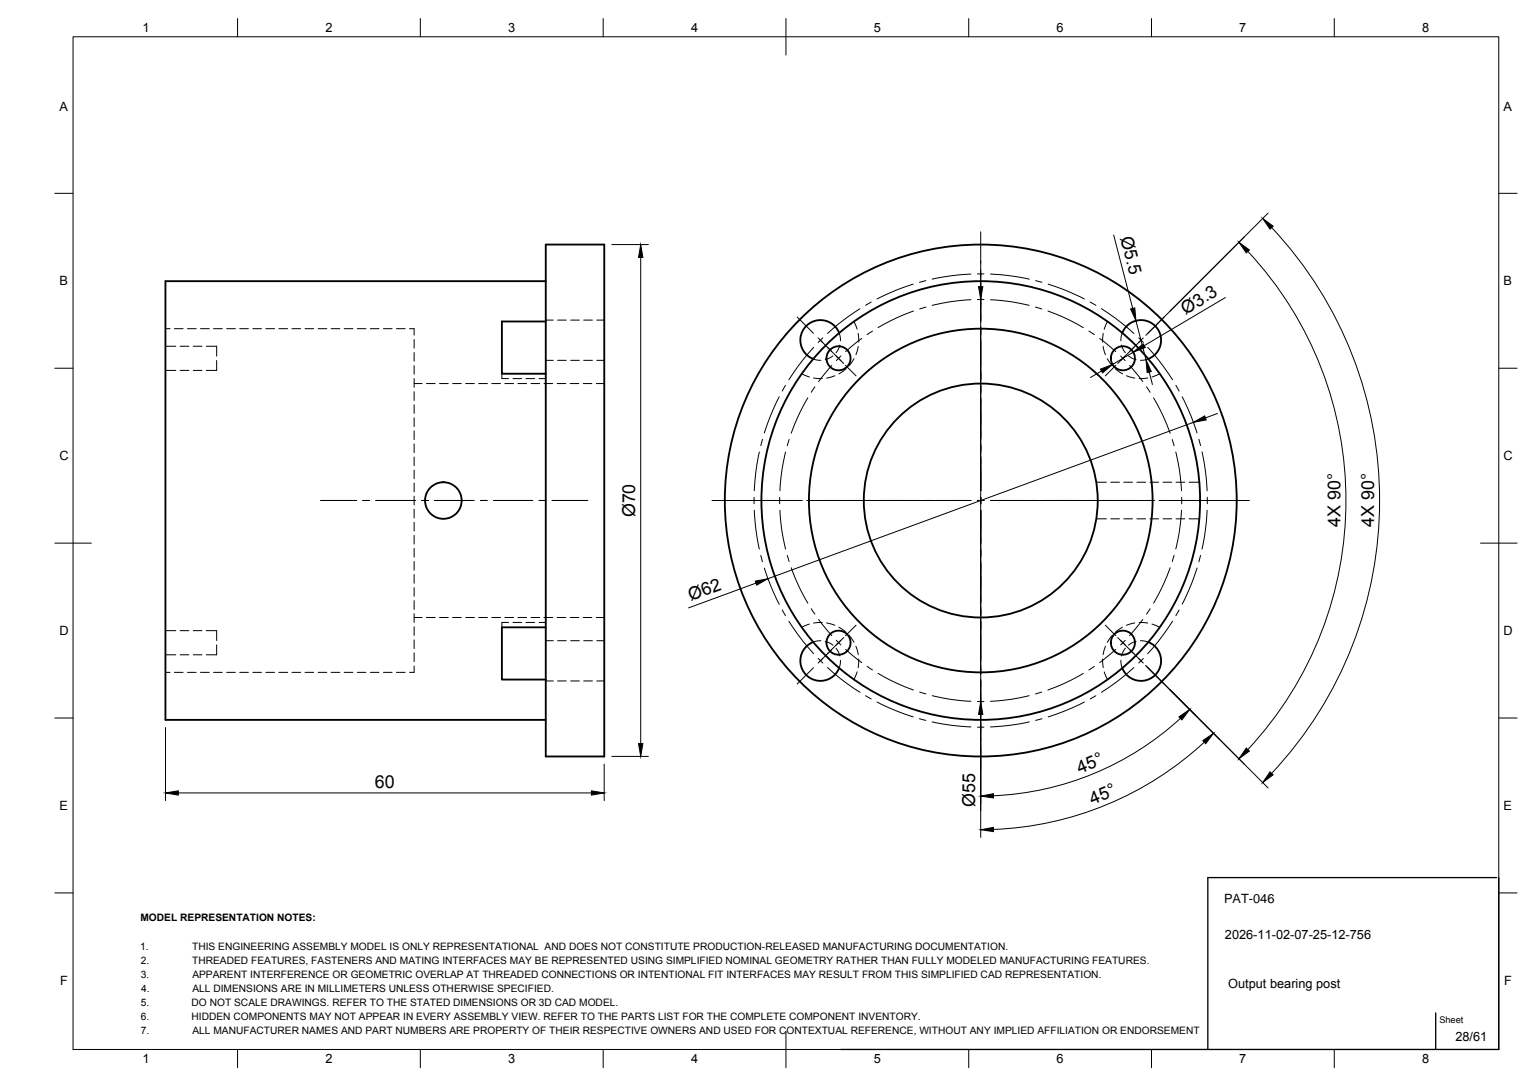
ISO-10303-21;
HEADER;
/* Generated by software containing ST-Developer
 * from STEP Tools, Inc. (www.steptools.com) 
 */

FILE_DESCRIPTION(
/* description */ ('Gear mesh backlash fixture'),
/* implementation_level */ '2;1');

FILE_NAME(
/* name */ 'Output bearing post.step',
/* time_stamp */ '2026-10-28T03:26:00-07:00',
/* author */ (''),
/* organization */ (''),
/* preprocessor_version */ 'ST-DEVELOPER v20.2',
/* originating_system */ 'Autodesk Translation Framework v15.17.0.0',
/* authorisation */ '');

FILE_SCHEMA (('AUTOMOTIVE_DESIGN { 1 0 10303 214 3 1 1 }'));
ENDSEC;

DATA;
#10=MECHANICAL_DESIGN_GEOMETRIC_PRESENTATION_REPRESENTATION('',(#1043),#57900);
#805=B_SPLINE_CURVE_WITH_KNOTS('',3,(#20786,#20787,#20788,#20789,#20790,
#20791,#20792,#20793,#20794,#20795),.UNSPECIFIED.,.F.,.F.,(4,2,2,2,4),(0.,
0.0943388977190341,0.188677795438068,0.283014752973434,0.377351710508801),
 .UNSPECIFIED.);
#806=B_SPLINE_CURVE_WITH_KNOTS('',3,(#20796,#20797,#20798,#20799,#20800,
#20801,#20802,#20803,#20804,#20805,#20806,#20807,#20808,#20809,#20810,#20811,
#20812,#20813,#20814,#20815,#20816,#20817,#20818,#20819,#20820,#20821),
 .UNSPECIFIED.,.F.,.F.,(4,2,2,2,2,2,2,2,2,2,2,2,4),(0.377351710508801,0.471688668044167,
0.566025625579534,0.660364523298568,0.754703421017602,0.849042318736636,
0.94338121645567,1.03771817399104,1.1320551315264,1.22639208906177,1.32072904659714,
1.41506794431617,1.5094068420352),.UNSPECIFIED.);
#807=B_SPLINE_CURVE_WITH_KNOTS('',3,(#20825,#20826,#20827,#20828,#20829,
#20830,#20831,#20832,#20833,#20834,#20835,#20836,#20837,#20838,#20839,#20840,
#20841,#20842,#20843,#20844,#20845,#20846,#20847,#20848,#20849,#20850),
 .UNSPECIFIED.,.F.,.F.,(4,2,2,2,2,2,2,2,2,2,2,2,4),(0.,0.0942186410044056,
0.188437282008811,0.282655768798836,0.376874255588861,0.471092742378886,
0.565311229168911,0.659529870173316,0.753748511177722,0.847967152182128,
0.942185793186533,1.03640427997656,1.13062276676658),.UNSPECIFIED.);
#808=B_SPLINE_CURVE_WITH_KNOTS('',3,(#20851,#20852,#20853,#20854,#20855,
#20856,#20857,#20858,#20859,#20860),.UNSPECIFIED.,.F.,.F.,(4,2,2,2,4),(1.13062276676658,
1.22484125355661,1.31905974034663,1.41327838135104,1.50749702235544),
 .UNSPECIFIED.);
#936=SHAPE_REPRESENTATION_RELATIONSHIP('SRR','None',#58133,#986);
#986=ADVANCED_BREP_SHAPE_REPRESENTATION('',(#1107),#57866);
#1043=STYLED_ITEM('',(#58465),#1107);
#1107=MANIFOLD_SOLID_BREP('Body1',#13604);
#1246=FACE_BOUND('',#2820,.T.);
#1247=FACE_BOUND('',#2821,.T.);
#1248=FACE_BOUND('',#2822,.T.);
#1249=FACE_BOUND('',#2823,.T.);
#1250=FACE_BOUND('',#2824,.T.);
#1251=FACE_BOUND('',#2829,.T.);
#1252=FACE_BOUND('',#2832,.T.);
#1253=FACE_BOUND('',#2835,.T.);
#1254=FACE_BOUND('',#2837,.T.);
#1255=FACE_BOUND('',#2838,.T.);
#1256=FACE_BOUND('',#2839,.T.);
#1257=FACE_BOUND('',#2840,.T.);
#1258=FACE_BOUND('',#2841,.T.);
#1259=FACE_BOUND('',#2843,.T.);
#1260=FACE_BOUND('',#2844,.T.);
#1261=FACE_BOUND('',#2845,.T.);
#1262=FACE_BOUND('',#2846,.T.);
#1263=FACE_BOUND('',#2847,.T.);
#1458=PLANE('',#14706);
#1459=PLANE('',#14710);
#1460=PLANE('',#14714);
#1461=PLANE('',#14718);
#1462=PLANE('',#14722);
#1463=PLANE('',#14727);
#1464=PLANE('',#14732);
#1465=PLANE('',#14737);
#1466=PLANE('',#14742);
#1467=PLANE('',#14763);
#1468=PLANE('',#14769);
#1469=PLANE('',#14770);
#1933=FACE_OUTER_BOUND('',#2801,.T.);
#1934=FACE_OUTER_BOUND('',#2802,.T.);
#1935=FACE_OUTER_BOUND('',#2803,.T.);
#1936=FACE_OUTER_BOUND('',#2804,.T.);
#1937=FACE_OUTER_BOUND('',#2805,.T.);
#1938=FACE_OUTER_BOUND('',#2806,.T.);
#1939=FACE_OUTER_BOUND('',#2807,.T.);
#1940=FACE_OUTER_BOUND('',#2808,.T.);
#1941=FACE_OUTER_BOUND('',#2809,.T.);
#1942=FACE_OUTER_BOUND('',#2810,.T.);
#1943=FACE_OUTER_BOUND('',#2811,.T.);
#1944=FACE_OUTER_BOUND('',#2812,.T.);
#1945=FACE_OUTER_BOUND('',#2813,.T.);
#1946=FACE_OUTER_BOUND('',#2814,.T.);
#1947=FACE_OUTER_BOUND('',#2815,.T.);
#1948=FACE_OUTER_BOUND('',#2816,.T.);
#1949=FACE_OUTER_BOUND('',#2817,.T.);
#1950=FACE_OUTER_BOUND('',#2818,.T.);
#1951=FACE_OUTER_BOUND('',#2819,.T.);
#1952=FACE_OUTER_BOUND('',#2825,.T.);
#1953=FACE_OUTER_BOUND('',#2826,.T.);
#1954=FACE_OUTER_BOUND('',#2827,.T.);
#1955=FACE_OUTER_BOUND('',#2828,.T.);
#1956=FACE_OUTER_BOUND('',#2830,.T.);
#1957=FACE_OUTER_BOUND('',#2831,.T.);
#1958=FACE_OUTER_BOUND('',#2833,.T.);
#1959=FACE_OUTER_BOUND('',#2834,.T.);
#1960=FACE_OUTER_BOUND('',#2836,.T.);
#1961=FACE_OUTER_BOUND('',#2842,.T.);
#2801=EDGE_LOOP('',(#9947,#9948,#9949,#9950,#9951,#9952));
#2802=EDGE_LOOP('',(#9953,#9954,#9955,#9956));
#2803=EDGE_LOOP('',(#9957));
#2804=EDGE_LOOP('',(#9958,#9959,#9960,#9961));
#2805=EDGE_LOOP('',(#9962));
#2806=EDGE_LOOP('',(#9963,#9964,#9965,#9966));
#2807=EDGE_LOOP('',(#9967));
#2808=EDGE_LOOP('',(#9968,#9969,#9970,#9971));
#2809=EDGE_LOOP('',(#9972));
#2810=EDGE_LOOP('',(#9973,#9974,#9975,#9976));
#2811=EDGE_LOOP('',(#9977,#9978));
#2812=EDGE_LOOP('',(#9979,#9980,#9981,#9982));
#2813=EDGE_LOOP('',(#9983,#9984));
#2814=EDGE_LOOP('',(#9985,#9986,#9987,#9988));
#2815=EDGE_LOOP('',(#9989,#9990));
#2816=EDGE_LOOP('',(#9991,#9992,#9993,#9994));
#2817=EDGE_LOOP('',(#9995,#9996));
#2818=EDGE_LOOP('',(#9997,#9998,#9999,#10000));
#2819=EDGE_LOOP('',(#10001));
#2820=EDGE_LOOP('',(#10002,#10003,#10004,#10005,#10006,#10007,#10008,#10009,
#10010));
#2821=EDGE_LOOP('',(#10011));
#2822=EDGE_LOOP('',(#10012));
#2823=EDGE_LOOP('',(#10013));
#2824=EDGE_LOOP('',(#10014));
#2825=EDGE_LOOP('',(#10015,#10016,#10017,#10018));
#2826=EDGE_LOOP('',(#10019,#10020,#10021,#10022));
#2827=EDGE_LOOP('',(#10023,#10024,#10025,#10026));
#2828=EDGE_LOOP('',(#10027,#10028,#10029,#10030,#10031,#10032,#10033,#10034,
#10035,#10036,#10037,#10038,#10039,#10040,#10041,#10042,#10043,#10044,#10045,
#10046));
#2829=EDGE_LOOP('',(#10047,#10048));
#2830=EDGE_LOOP('',(#10049,#10050,#10051,#10052));
#2831=EDGE_LOOP('',(#10053));
#2832=EDGE_LOOP('',(#10054));
#2833=EDGE_LOOP('',(#10055,#10056,#10057,#10058));
#2834=EDGE_LOOP('',(#10059,#10060,#10061,#10062));
#2835=EDGE_LOOP('',(#10063,#10064));
#2836=EDGE_LOOP('',(#10065));
#2837=EDGE_LOOP('',(#10066));
#2838=EDGE_LOOP('',(#10067));
#2839=EDGE_LOOP('',(#10068));
#2840=EDGE_LOOP('',(#10069));
#2841=EDGE_LOOP('',(#10070));
#2842=EDGE_LOOP('',(#10071));
#2843=EDGE_LOOP('',(#10072));
#2844=EDGE_LOOP('',(#10073));
#2845=EDGE_LOOP('',(#10074));
#2846=EDGE_LOOP('',(#10075));
#2847=EDGE_LOOP('',(#10076));
#3686=LINE('',#20823,#4575);
#3687=LINE('',#20865,#4576);
#3688=LINE('',#20872,#4577);
#3689=LINE('',#20879,#4578);
#3690=LINE('',#20886,#4579);
#3691=LINE('',#20892,#4580);
#3692=LINE('',#20896,#4581);
#3693=LINE('',#20903,#4582);
#3694=LINE('',#20907,#4583);
#3695=LINE('',#20914,#4584);
#3696=LINE('',#20918,#4585);
#3697=LINE('',#20925,#4586);
#3698=LINE('',#20929,#4587);
#3699=LINE('',#20937,#4588);
#3700=LINE('',#20957,#4589);
#3701=LINE('',#20961,#4590);
#3702=LINE('',#20965,#4591);
#3703=LINE('',#20969,#4592);
#3704=LINE('',#20974,#4593);
#3705=LINE('',#20981,#4594);
#3706=LINE('',#20985,#4595);
#4575=VECTOR('',#16869,0.25);
#4576=VECTOR('',#16874,0.165);
#4577=VECTOR('',#16883,0.165);
#4578=VECTOR('',#16892,0.164999999999999);
#4579=VECTOR('',#16901,0.165);
#4580=VECTOR('',#16908,1.);
#4581=VECTOR('',#16911,1.);
#4582=VECTOR('',#16920,1.);
#4583=VECTOR('',#16923,1.);
#4584=VECTOR('',#16932,1.);
#4585=VECTOR('',#16935,1.);
#4586=VECTOR('',#16944,1.);
#4587=VECTOR('',#16947,1.);
#4588=VECTOR('',#16958,0.275);
#4589=VECTOR('',#16985,0.275);
#4590=VECTOR('',#16990,0.275);
#4591=VECTOR('',#16995,0.275);
#4592=VECTOR('',#17000,3.);
#4593=VECTOR('',#17005,2.35);
#4594=VECTOR('',#17014,3.5);
#4595=VECTOR('',#17019,1.6);
#5427=CIRCLE('',#14704,0.165);
#5428=CIRCLE('',#14705,0.165);
#5429=CIRCLE('',#14708,0.165);
#5430=CIRCLE('',#14709,0.165);
#5431=CIRCLE('',#14712,0.164999999999999);
#5432=CIRCLE('',#14713,0.164999999999999);
#5433=CIRCLE('',#14716,0.165);
#5434=CIRCLE('',#14717,0.165);
#5435=CIRCLE('',#14720,0.525);
#5436=CIRCLE('',#14721,0.525);
#5437=CIRCLE('',#14723,3.);
#5438=CIRCLE('',#14725,0.525);
#5439=CIRCLE('',#14726,0.525);
#5440=CIRCLE('',#14728,3.);
#5441=CIRCLE('',#14730,0.525);
#5442=CIRCLE('',#14731,0.525);
#5443=CIRCLE('',#14733,3.);
#5444=CIRCLE('',#14735,0.525);
#5445=CIRCLE('',#14736,0.525);
#5446=CIRCLE('',#14738,3.);
#5447=CIRCLE('',#14740,0.275);
#5448=CIRCLE('',#14741,0.275);
#5449=CIRCLE('',#14743,3.5);
#5450=CIRCLE('',#14744,3.);
#5451=CIRCLE('',#14745,3.);
#5452=CIRCLE('',#14746,3.);
#5453=CIRCLE('',#14747,3.);
#5454=CIRCLE('',#14748,3.);
#5455=CIRCLE('',#14749,0.275);
#5456=CIRCLE('',#14750,0.275);
#5457=CIRCLE('',#14751,0.275);
#5458=CIRCLE('',#14753,0.275);
#5459=CIRCLE('',#14755,0.275);
#5460=CIRCLE('',#14757,0.275);
#5461=CIRCLE('',#14759,3.);
#5462=CIRCLE('',#14761,2.35);
#5463=CIRCLE('',#14762,2.35);
#5464=CIRCLE('',#14764,1.6);
#5465=CIRCLE('',#14766,3.5);
#5466=CIRCLE('',#14768,1.6);
#6139=VERTEX_POINT('',#20784);
#6140=VERTEX_POINT('',#20785);
#6141=VERTEX_POINT('',#20822);
#6142=VERTEX_POINT('',#20824);
#6143=VERTEX_POINT('',#20862);
#6144=VERTEX_POINT('',#20864);
#6145=VERTEX_POINT('',#20869);
#6146=VERTEX_POINT('',#20871);
#6147=VERTEX_POINT('',#20876);
#6148=VERTEX_POINT('',#20878);
#6149=VERTEX_POINT('',#20883);
#6150=VERTEX_POINT('',#20885);
#6151=VERTEX_POINT('',#20890);
#6152=VERTEX_POINT('',#20891);
#6153=VERTEX_POINT('',#20893);
#6154=VERTEX_POINT('',#20895);
#6155=VERTEX_POINT('',#20901);
#6156=VERTEX_POINT('',#20902);
#6157=VERTEX_POINT('',#20904);
#6158=VERTEX_POINT('',#20906);
#6159=VERTEX_POINT('',#20912);
#6160=VERTEX_POINT('',#20913);
#6161=VERTEX_POINT('',#20915);
#6162=VERTEX_POINT('',#20917);
#6163=VERTEX_POINT('',#20923);
#6164=VERTEX_POINT('',#20924);
#6165=VERTEX_POINT('',#20926);
#6166=VERTEX_POINT('',#20928);
#6167=VERTEX_POINT('',#20934);
#6168=VERTEX_POINT('',#20936);
#6169=VERTEX_POINT('',#20940);
#6170=VERTEX_POINT('',#20942);
#6171=VERTEX_POINT('',#20948);
#6172=VERTEX_POINT('',#20950);
#6173=VERTEX_POINT('',#20952);
#6174=VERTEX_POINT('',#20955);
#6175=VERTEX_POINT('',#20959);
#6176=VERTEX_POINT('',#20963);
#6177=VERTEX_POINT('',#20967);
#6178=VERTEX_POINT('',#20971);
#6179=VERTEX_POINT('',#20973);
#6180=VERTEX_POINT('',#20977);
#6181=VERTEX_POINT('',#20980);
#6182=VERTEX_POINT('',#20984);
#7560=EDGE_CURVE('',#6139,#6140,#805,.T.);
#7561=EDGE_CURVE('',#6140,#6139,#806,.T.);
#7562=EDGE_CURVE('',#6140,#6141,#3686,.T.);
#7563=EDGE_CURVE('',#6142,#6141,#807,.T.);
#7564=EDGE_CURVE('',#6141,#6142,#808,.T.);
#7565=EDGE_CURVE('',#6143,#6143,#5427,.T.);
#7566=EDGE_CURVE('',#6143,#6144,#3687,.T.);
#7567=EDGE_CURVE('',#6144,#6144,#5428,.T.);
#7568=EDGE_CURVE('',#6145,#6145,#5429,.T.);
#7569=EDGE_CURVE('',#6145,#6146,#3688,.T.);
#7570=EDGE_CURVE('',#6146,#6146,#5430,.T.);
#7571=EDGE_CURVE('',#6147,#6147,#5431,.T.);
#7572=EDGE_CURVE('',#6147,#6148,#3689,.T.);
#7573=EDGE_CURVE('',#6148,#6148,#5432,.T.);
#7574=EDGE_CURVE('',#6149,#6149,#5433,.T.);
#7575=EDGE_CURVE('',#6149,#6150,#3690,.T.);
#7576=EDGE_CURVE('',#6150,#6150,#5434,.T.);
#7577=EDGE_CURVE('',#6151,#6152,#3691,.T.);
#7578=EDGE_CURVE('',#6151,#6153,#5435,.T.);
#7579=EDGE_CURVE('',#6154,#6153,#3692,.T.);
#7580=EDGE_CURVE('',#6152,#6154,#5436,.T.);
#7581=EDGE_CURVE('',#6153,#6151,#5437,.T.);
#7582=EDGE_CURVE('',#6155,#6156,#3693,.T.);
#7583=EDGE_CURVE('',#6155,#6157,#5438,.T.);
#7584=EDGE_CURVE('',#6158,#6157,#3694,.T.);
#7585=EDGE_CURVE('',#6156,#6158,#5439,.T.);
#7586=EDGE_CURVE('',#6157,#6155,#5440,.T.);
#7587=EDGE_CURVE('',#6159,#6160,#3695,.T.);
#7588=EDGE_CURVE('',#6159,#6161,#5441,.T.);
#7589=EDGE_CURVE('',#6162,#6161,#3696,.T.);
#7590=EDGE_CURVE('',#6160,#6162,#5442,.T.);
#7591=EDGE_CURVE('',#6161,#6159,#5443,.T.);
#7592=EDGE_CURVE('',#6163,#6164,#3697,.T.);
#7593=EDGE_CURVE('',#6163,#6165,#5444,.T.);
#7594=EDGE_CURVE('',#6166,#6165,#3698,.T.);
#7595=EDGE_CURVE('',#6164,#6166,#5445,.T.);
#7596=EDGE_CURVE('',#6165,#6163,#5446,.T.);
#7597=EDGE_CURVE('',#6167,#6167,#5447,.T.);
#7598=EDGE_CURVE('',#6167,#6168,#3699,.T.);
#7599=EDGE_CURVE('',#6168,#6168,#5448,.T.);
#7600=EDGE_CURVE('',#6169,#6169,#5449,.T.);
#7601=EDGE_CURVE('',#6156,#6170,#5450,.T.);
#7602=EDGE_CURVE('',#6160,#6158,#5451,.T.);
#7603=EDGE_CURVE('',#6164,#6162,#5452,.T.);
#7604=EDGE_CURVE('',#6152,#6166,#5453,.T.);
#7605=EDGE_CURVE('',#6170,#6154,#5454,.T.);
#7606=EDGE_CURVE('',#6171,#6171,#5455,.T.);
#7607=EDGE_CURVE('',#6172,#6172,#5456,.T.);
#7608=EDGE_CURVE('',#6173,#6173,#5457,.T.);
#7609=EDGE_CURVE('',#6174,#6174,#5458,.T.);
#7610=EDGE_CURVE('',#6174,#6172,#3700,.T.);
#7611=EDGE_CURVE('',#6175,#6175,#5459,.T.);
#7612=EDGE_CURVE('',#6175,#6171,#3701,.T.);
#7613=EDGE_CURVE('',#6176,#6176,#5460,.T.);
#7614=EDGE_CURVE('',#6176,#6173,#3702,.T.);
#7615=EDGE_CURVE('',#6177,#6177,#5461,.T.);
#7616=EDGE_CURVE('',#6177,#6170,#3703,.T.);
#7617=EDGE_CURVE('',#6178,#6178,#5462,.T.);
#7618=EDGE_CURVE('',#6178,#6179,#3704,.T.);
#7619=EDGE_CURVE('',#6179,#6179,#5463,.T.);
#7620=EDGE_CURVE('',#6180,#6180,#5464,.T.);
#7621=EDGE_CURVE('',#6169,#6181,#3705,.T.);
#7622=EDGE_CURVE('',#6181,#6181,#5465,.T.);
#7623=EDGE_CURVE('',#6180,#6182,#3706,.T.);
#7624=EDGE_CURVE('',#6182,#6182,#5466,.T.);
#9947=ORIENTED_EDGE('',*,*,#7560,.F.);
#9948=ORIENTED_EDGE('',*,*,#7561,.F.);
#9949=ORIENTED_EDGE('',*,*,#7562,.T.);
#9950=ORIENTED_EDGE('',*,*,#7563,.F.);
#9951=ORIENTED_EDGE('',*,*,#7564,.F.);
#9952=ORIENTED_EDGE('',*,*,#7562,.F.);
#9953=ORIENTED_EDGE('',*,*,#7565,.F.);
#9954=ORIENTED_EDGE('',*,*,#7566,.T.);
#9955=ORIENTED_EDGE('',*,*,#7567,.F.);
#9956=ORIENTED_EDGE('',*,*,#7566,.F.);
#9957=ORIENTED_EDGE('',*,*,#7565,.T.);
#9958=ORIENTED_EDGE('',*,*,#7568,.F.);
#9959=ORIENTED_EDGE('',*,*,#7569,.T.);
#9960=ORIENTED_EDGE('',*,*,#7570,.F.);
#9961=ORIENTED_EDGE('',*,*,#7569,.F.);
#9962=ORIENTED_EDGE('',*,*,#7568,.T.);
#9963=ORIENTED_EDGE('',*,*,#7571,.F.);
#9964=ORIENTED_EDGE('',*,*,#7572,.T.);
#9965=ORIENTED_EDGE('',*,*,#7573,.F.);
#9966=ORIENTED_EDGE('',*,*,#7572,.F.);
#9967=ORIENTED_EDGE('',*,*,#7571,.T.);
#9968=ORIENTED_EDGE('',*,*,#7574,.F.);
#9969=ORIENTED_EDGE('',*,*,#7575,.T.);
#9970=ORIENTED_EDGE('',*,*,#7576,.F.);
#9971=ORIENTED_EDGE('',*,*,#7575,.F.);
#9972=ORIENTED_EDGE('',*,*,#7574,.T.);
#9973=ORIENTED_EDGE('',*,*,#7577,.F.);
#9974=ORIENTED_EDGE('',*,*,#7578,.T.);
#9975=ORIENTED_EDGE('',*,*,#7579,.F.);
#9976=ORIENTED_EDGE('',*,*,#7580,.F.);
#9977=ORIENTED_EDGE('',*,*,#7581,.F.);
#9978=ORIENTED_EDGE('',*,*,#7578,.F.);
#9979=ORIENTED_EDGE('',*,*,#7582,.F.);
#9980=ORIENTED_EDGE('',*,*,#7583,.T.);
#9981=ORIENTED_EDGE('',*,*,#7584,.F.);
#9982=ORIENTED_EDGE('',*,*,#7585,.F.);
#9983=ORIENTED_EDGE('',*,*,#7586,.F.);
#9984=ORIENTED_EDGE('',*,*,#7583,.F.);
#9985=ORIENTED_EDGE('',*,*,#7587,.F.);
#9986=ORIENTED_EDGE('',*,*,#7588,.T.);
#9987=ORIENTED_EDGE('',*,*,#7589,.F.);
#9988=ORIENTED_EDGE('',*,*,#7590,.F.);
#9989=ORIENTED_EDGE('',*,*,#7591,.F.);
#9990=ORIENTED_EDGE('',*,*,#7588,.F.);
#9991=ORIENTED_EDGE('',*,*,#7592,.F.);
#9992=ORIENTED_EDGE('',*,*,#7593,.T.);
#9993=ORIENTED_EDGE('',*,*,#7594,.F.);
#9994=ORIENTED_EDGE('',*,*,#7595,.F.);
#9995=ORIENTED_EDGE('',*,*,#7596,.F.);
#9996=ORIENTED_EDGE('',*,*,#7593,.F.);
#9997=ORIENTED_EDGE('',*,*,#7597,.F.);
#9998=ORIENTED_EDGE('',*,*,#7598,.T.);
#9999=ORIENTED_EDGE('',*,*,#7599,.F.);
#10000=ORIENTED_EDGE('',*,*,#7598,.F.);
#10001=ORIENTED_EDGE('',*,*,#7600,.T.);
#10002=ORIENTED_EDGE('',*,*,#7601,.F.);
#10003=ORIENTED_EDGE('',*,*,#7585,.T.);
#10004=ORIENTED_EDGE('',*,*,#7602,.F.);
#10005=ORIENTED_EDGE('',*,*,#7590,.T.);
#10006=ORIENTED_EDGE('',*,*,#7603,.F.);
#10007=ORIENTED_EDGE('',*,*,#7595,.T.);
#10008=ORIENTED_EDGE('',*,*,#7604,.F.);
#10009=ORIENTED_EDGE('',*,*,#7580,.T.);
#10010=ORIENTED_EDGE('',*,*,#7605,.F.);
#10011=ORIENTED_EDGE('',*,*,#7606,.T.);
#10012=ORIENTED_EDGE('',*,*,#7599,.T.);
#10013=ORIENTED_EDGE('',*,*,#7607,.T.);
#10014=ORIENTED_EDGE('',*,*,#7608,.T.);
#10015=ORIENTED_EDGE('',*,*,#7609,.F.);
#10016=ORIENTED_EDGE('',*,*,#7610,.T.);
#10017=ORIENTED_EDGE('',*,*,#7607,.F.);
#10018=ORIENTED_EDGE('',*,*,#7610,.F.);
#10019=ORIENTED_EDGE('',*,*,#7611,.F.);
#10020=ORIENTED_EDGE('',*,*,#7612,.T.);
#10021=ORIENTED_EDGE('',*,*,#7606,.F.);
#10022=ORIENTED_EDGE('',*,*,#7612,.F.);
#10023=ORIENTED_EDGE('',*,*,#7613,.F.);
#10024=ORIENTED_EDGE('',*,*,#7614,.T.);
#10025=ORIENTED_EDGE('',*,*,#7608,.F.);
#10026=ORIENTED_EDGE('',*,*,#7614,.F.);
#10027=ORIENTED_EDGE('',*,*,#7615,.F.);
#10028=ORIENTED_EDGE('',*,*,#7616,.T.);
#10029=ORIENTED_EDGE('',*,*,#7605,.T.);
#10030=ORIENTED_EDGE('',*,*,#7579,.T.);
#10031=ORIENTED_EDGE('',*,*,#7581,.T.);
#10032=ORIENTED_EDGE('',*,*,#7577,.T.);
#10033=ORIENTED_EDGE('',*,*,#7604,.T.);
#10034=ORIENTED_EDGE('',*,*,#7594,.T.);
#10035=ORIENTED_EDGE('',*,*,#7596,.T.);
#10036=ORIENTED_EDGE('',*,*,#7592,.T.);
#10037=ORIENTED_EDGE('',*,*,#7603,.T.);
#10038=ORIENTED_EDGE('',*,*,#7589,.T.);
#10039=ORIENTED_EDGE('',*,*,#7591,.T.);
#10040=ORIENTED_EDGE('',*,*,#7587,.T.);
#10041=ORIENTED_EDGE('',*,*,#7602,.T.);
#10042=ORIENTED_EDGE('',*,*,#7584,.T.);
#10043=ORIENTED_EDGE('',*,*,#7586,.T.);
#10044=ORIENTED_EDGE('',*,*,#7582,.T.);
#10045=ORIENTED_EDGE('',*,*,#7601,.T.);
#10046=ORIENTED_EDGE('',*,*,#7616,.F.);
#10047=ORIENTED_EDGE('',*,*,#7563,.T.);
#10048=ORIENTED_EDGE('',*,*,#7564,.T.);
#10049=ORIENTED_EDGE('',*,*,#7617,.F.);
#10050=ORIENTED_EDGE('',*,*,#7618,.T.);
#10051=ORIENTED_EDGE('',*,*,#7619,.F.);
#10052=ORIENTED_EDGE('',*,*,#7618,.F.);
#10053=ORIENTED_EDGE('',*,*,#7617,.T.);
#10054=ORIENTED_EDGE('',*,*,#7620,.F.);
#10055=ORIENTED_EDGE('',*,*,#7600,.F.);
#10056=ORIENTED_EDGE('',*,*,#7621,.T.);
#10057=ORIENTED_EDGE('',*,*,#7622,.T.);
#10058=ORIENTED_EDGE('',*,*,#7621,.F.);
#10059=ORIENTED_EDGE('',*,*,#7620,.T.);
#10060=ORIENTED_EDGE('',*,*,#7623,.T.);
#10061=ORIENTED_EDGE('',*,*,#7624,.T.);
#10062=ORIENTED_EDGE('',*,*,#7623,.F.);
#10063=ORIENTED_EDGE('',*,*,#7560,.T.);
#10064=ORIENTED_EDGE('',*,*,#7561,.T.);
#10065=ORIENTED_EDGE('',*,*,#7615,.T.);
#10066=ORIENTED_EDGE('',*,*,#7619,.T.);
#10067=ORIENTED_EDGE('',*,*,#7576,.T.);
#10068=ORIENTED_EDGE('',*,*,#7573,.T.);
#10069=ORIENTED_EDGE('',*,*,#7570,.T.);
#10070=ORIENTED_EDGE('',*,*,#7567,.T.);
#10071=ORIENTED_EDGE('',*,*,#7622,.F.);
#10072=ORIENTED_EDGE('',*,*,#7624,.F.);
#10073=ORIENTED_EDGE('',*,*,#7609,.T.);
#10074=ORIENTED_EDGE('',*,*,#7597,.T.);
#10075=ORIENTED_EDGE('',*,*,#7613,.T.);
#10076=ORIENTED_EDGE('',*,*,#7611,.T.);
#12672=CYLINDRICAL_SURFACE('',#14702,0.25);
#12673=CYLINDRICAL_SURFACE('',#14703,0.165);
#12674=CYLINDRICAL_SURFACE('',#14707,0.165);
#12675=CYLINDRICAL_SURFACE('',#14711,0.164999999999999);
#12676=CYLINDRICAL_SURFACE('',#14715,0.165);
#12677=CYLINDRICAL_SURFACE('',#14719,0.525);
#12678=CYLINDRICAL_SURFACE('',#14724,0.525);
#12679=CYLINDRICAL_SURFACE('',#14729,0.525);
#12680=CYLINDRICAL_SURFACE('',#14734,0.525);
#12681=CYLINDRICAL_SURFACE('',#14739,0.275);
#12682=CYLINDRICAL_SURFACE('',#14752,0.275);
#12683=CYLINDRICAL_SURFACE('',#14754,0.275);
#12684=CYLINDRICAL_SURFACE('',#14756,0.275);
#12685=CYLINDRICAL_SURFACE('',#14758,3.);
#12686=CYLINDRICAL_SURFACE('',#14760,2.35);
#12687=CYLINDRICAL_SURFACE('',#14765,3.5);
#12688=CYLINDRICAL_SURFACE('',#14767,1.6);
#13050=ADVANCED_FACE('',(#1933),#12672,.F.);
#13051=ADVANCED_FACE('',(#1934),#12673,.F.);
#13052=ADVANCED_FACE('',(#1935),#1458,.T.);
#13053=ADVANCED_FACE('',(#1936),#12674,.F.);
#13054=ADVANCED_FACE('',(#1937),#1459,.T.);
#13055=ADVANCED_FACE('',(#1938),#12675,.F.);
#13056=ADVANCED_FACE('',(#1939),#1460,.T.);
#13057=ADVANCED_FACE('',(#1940),#12676,.F.);
#13058=ADVANCED_FACE('',(#1941),#1461,.T.);
#13059=ADVANCED_FACE('',(#1942),#12677,.F.);
#13060=ADVANCED_FACE('',(#1943),#1462,.F.);
#13061=ADVANCED_FACE('',(#1944),#12678,.F.);
#13062=ADVANCED_FACE('',(#1945),#1463,.F.);
#13063=ADVANCED_FACE('',(#1946),#12679,.F.);
#13064=ADVANCED_FACE('',(#1947),#1464,.F.);
#13065=ADVANCED_FACE('',(#1948),#12680,.F.);
#13066=ADVANCED_FACE('',(#1949),#1465,.F.);
#13067=ADVANCED_FACE('',(#1950),#12681,.F.);
#13068=ADVANCED_FACE('',(#1951,#1246,#1247,#1248,#1249,#1250),#1466,.T.);
#13069=ADVANCED_FACE('',(#1952),#12682,.F.);
#13070=ADVANCED_FACE('',(#1953),#12683,.F.);
#13071=ADVANCED_FACE('',(#1954),#12684,.F.);
#13072=ADVANCED_FACE('',(#1955,#1251),#12685,.T.);
#13073=ADVANCED_FACE('',(#1956),#12686,.F.);
#13074=ADVANCED_FACE('',(#1957,#1252),#1467,.T.);
#13075=ADVANCED_FACE('',(#1958),#12687,.T.);
#13076=ADVANCED_FACE('',(#1959,#1253),#12688,.F.);
#13077=ADVANCED_FACE('',(#1960,#1254,#1255,#1256,#1257,#1258),#1468,.T.);
#13078=ADVANCED_FACE('',(#1961,#1259,#1260,#1261,#1262,#1263),#1469,.F.);
#13604=CLOSED_SHELL('',(#13050,#13051,#13052,#13053,#13054,#13055,#13056,
#13057,#13058,#13059,#13060,#13061,#13062,#13063,#13064,#13065,#13066,#13067,
#13068,#13069,#13070,#13071,#13072,#13073,#13074,#13075,#13076,#13077,#13078));
#14701=AXIS2_PLACEMENT_3D('',#20782,#16865,#16866);
#14702=AXIS2_PLACEMENT_3D('',#20783,#16867,#16868);
#14703=AXIS2_PLACEMENT_3D('',#20861,#16870,#16871);
#14704=AXIS2_PLACEMENT_3D('',#20863,#16872,#16873);
#14705=AXIS2_PLACEMENT_3D('',#20866,#16875,#16876);
#14706=AXIS2_PLACEMENT_3D('',#20867,#16877,#16878);
#14707=AXIS2_PLACEMENT_3D('',#20868,#16879,#16880);
#14708=AXIS2_PLACEMENT_3D('',#20870,#16881,#16882);
#14709=AXIS2_PLACEMENT_3D('',#20873,#16884,#16885);
#14710=AXIS2_PLACEMENT_3D('',#20874,#16886,#16887);
#14711=AXIS2_PLACEMENT_3D('',#20875,#16888,#16889);
#14712=AXIS2_PLACEMENT_3D('',#20877,#16890,#16891);
#14713=AXIS2_PLACEMENT_3D('',#20880,#16893,#16894);
#14714=AXIS2_PLACEMENT_3D('',#20881,#16895,#16896);
#14715=AXIS2_PLACEMENT_3D('',#20882,#16897,#16898);
#14716=AXIS2_PLACEMENT_3D('',#20884,#16899,#16900);
#14717=AXIS2_PLACEMENT_3D('',#20887,#16902,#16903);
#14718=AXIS2_PLACEMENT_3D('',#20888,#16904,#16905);
#14719=AXIS2_PLACEMENT_3D('',#20889,#16906,#16907);
#14720=AXIS2_PLACEMENT_3D('',#20894,#16909,#16910);
#14721=AXIS2_PLACEMENT_3D('',#20897,#16912,#16913);
#14722=AXIS2_PLACEMENT_3D('',#20898,#16914,#16915);
#14723=AXIS2_PLACEMENT_3D('',#20899,#16916,#16917);
#14724=AXIS2_PLACEMENT_3D('',#20900,#16918,#16919);
#14725=AXIS2_PLACEMENT_3D('',#20905,#16921,#16922);
#14726=AXIS2_PLACEMENT_3D('',#20908,#16924,#16925);
#14727=AXIS2_PLACEMENT_3D('',#20909,#16926,#16927);
#14728=AXIS2_PLACEMENT_3D('',#20910,#16928,#16929);
#14729=AXIS2_PLACEMENT_3D('',#20911,#16930,#16931);
#14730=AXIS2_PLACEMENT_3D('',#20916,#16933,#16934);
#14731=AXIS2_PLACEMENT_3D('',#20919,#16936,#16937);
#14732=AXIS2_PLACEMENT_3D('',#20920,#16938,#16939);
#14733=AXIS2_PLACEMENT_3D('',#20921,#16940,#16941);
#14734=AXIS2_PLACEMENT_3D('',#20922,#16942,#16943);
#14735=AXIS2_PLACEMENT_3D('',#20927,#16945,#16946);
#14736=AXIS2_PLACEMENT_3D('',#20930,#16948,#16949);
#14737=AXIS2_PLACEMENT_3D('',#20931,#16950,#16951);
#14738=AXIS2_PLACEMENT_3D('',#20932,#16952,#16953);
#14739=AXIS2_PLACEMENT_3D('',#20933,#16954,#16955);
#14740=AXIS2_PLACEMENT_3D('',#20935,#16956,#16957);
#14741=AXIS2_PLACEMENT_3D('',#20938,#16959,#16960);
#14742=AXIS2_PLACEMENT_3D('',#20939,#16961,#16962);
#14743=AXIS2_PLACEMENT_3D('',#20941,#16963,#16964);
#14744=AXIS2_PLACEMENT_3D('',#20943,#16965,#16966);
#14745=AXIS2_PLACEMENT_3D('',#20944,#16967,#16968);
#14746=AXIS2_PLACEMENT_3D('',#20945,#16969,#16970);
#14747=AXIS2_PLACEMENT_3D('',#20946,#16971,#16972);
#14748=AXIS2_PLACEMENT_3D('',#20947,#16973,#16974);
#14749=AXIS2_PLACEMENT_3D('',#20949,#16975,#16976);
#14750=AXIS2_PLACEMENT_3D('',#20951,#16977,#16978);
#14751=AXIS2_PLACEMENT_3D('',#20953,#16979,#16980);
#14752=AXIS2_PLACEMENT_3D('',#20954,#16981,#16982);
#14753=AXIS2_PLACEMENT_3D('',#20956,#16983,#16984);
#14754=AXIS2_PLACEMENT_3D('',#20958,#16986,#16987);
#14755=AXIS2_PLACEMENT_3D('',#20960,#16988,#16989);
#14756=AXIS2_PLACEMENT_3D('',#20962,#16991,#16992);
#14757=AXIS2_PLACEMENT_3D('',#20964,#16993,#16994);
#14758=AXIS2_PLACEMENT_3D('',#20966,#16996,#16997);
#14759=AXIS2_PLACEMENT_3D('',#20968,#16998,#16999);
#14760=AXIS2_PLACEMENT_3D('',#20970,#17001,#17002);
#14761=AXIS2_PLACEMENT_3D('',#20972,#17003,#17004);
#14762=AXIS2_PLACEMENT_3D('',#20975,#17006,#17007);
#14763=AXIS2_PLACEMENT_3D('',#20976,#17008,#17009);
#14764=AXIS2_PLACEMENT_3D('',#20978,#17010,#17011);
#14765=AXIS2_PLACEMENT_3D('',#20979,#17012,#17013);
#14766=AXIS2_PLACEMENT_3D('',#20982,#17015,#17016);
#14767=AXIS2_PLACEMENT_3D('',#20983,#17017,#17018);
#14768=AXIS2_PLACEMENT_3D('',#20986,#17020,#17021);
#14769=AXIS2_PLACEMENT_3D('',#20987,#17022,#17023);
#14770=AXIS2_PLACEMENT_3D('',#20988,#17024,#17025);
#16865=DIRECTION('axis',(0.,0.,1.));
#16866=DIRECTION('refdir',(1.,0.,0.));
#16867=DIRECTION('center_axis',(1.,0.,0.));
#16868=DIRECTION('ref_axis',(0.,0.,-1.));
#16869=DIRECTION('',(1.,0.,0.));
#16870=DIRECTION('center_axis',(0.,0.,1.));
#16871=DIRECTION('ref_axis',(1.,0.,0.));
#16872=DIRECTION('center_axis',(0.,0.,1.));
#16873=DIRECTION('ref_axis',(1.,0.,0.));
#16874=DIRECTION('',(0.,0.,1.));
#16875=DIRECTION('center_axis',(0.,0.,-1.));
#16876=DIRECTION('ref_axis',(1.,0.,0.));
#16877=DIRECTION('center_axis',(0.,0.,1.));
#16878=DIRECTION('ref_axis',(1.,0.,0.));
#16879=DIRECTION('center_axis',(0.,0.,1.));
#16880=DIRECTION('ref_axis',(1.,0.,0.));
#16881=DIRECTION('center_axis',(0.,0.,1.));
#16882=DIRECTION('ref_axis',(1.,0.,0.));
#16883=DIRECTION('',(0.,0.,1.));
#16884=DIRECTION('center_axis',(0.,0.,-1.));
#16885=DIRECTION('ref_axis',(1.,0.,0.));
#16886=DIRECTION('center_axis',(0.,0.,1.));
#16887=DIRECTION('ref_axis',(1.,0.,0.));
#16888=DIRECTION('center_axis',(0.,0.,1.));
#16889=DIRECTION('ref_axis',(1.,0.,0.));
#16890=DIRECTION('center_axis',(0.,0.,1.));
#16891=DIRECTION('ref_axis',(1.,0.,0.));
#16892=DIRECTION('',(0.,0.,1.));
#16893=DIRECTION('center_axis',(0.,0.,-1.));
#16894=DIRECTION('ref_axis',(1.,0.,0.));
#16895=DIRECTION('center_axis',(0.,0.,1.));
#16896=DIRECTION('ref_axis',(1.,0.,0.));
#16897=DIRECTION('center_axis',(0.,0.,1.));
#16898=DIRECTION('ref_axis',(1.,0.,0.));
#16899=DIRECTION('center_axis',(0.,0.,1.));
#16900=DIRECTION('ref_axis',(1.,0.,0.));
#16901=DIRECTION('',(0.,0.,1.));
#16902=DIRECTION('center_axis',(0.,0.,-1.));
#16903=DIRECTION('ref_axis',(1.,0.,0.));
#16904=DIRECTION('center_axis',(0.,0.,1.));
#16905=DIRECTION('ref_axis',(1.,0.,0.));
#16906=DIRECTION('center_axis',(0.,0.,1.));
#16907=DIRECTION('ref_axis',(1.,0.,0.));
#16908=DIRECTION('',(0.,0.,-1.));
#16909=DIRECTION('center_axis',(0.,0.,1.));
#16910=DIRECTION('ref_axis',(1.,0.,0.));
#16911=DIRECTION('',(0.,0.,1.));
#16912=DIRECTION('center_axis',(0.,0.,1.));
#16913=DIRECTION('ref_axis',(1.,0.,0.));
#16914=DIRECTION('center_axis',(0.,0.,1.));
#16915=DIRECTION('ref_axis',(1.,0.,0.));
#16916=DIRECTION('center_axis',(0.,0.,1.));
#16917=DIRECTION('ref_axis',(1.,0.,0.));
#16918=DIRECTION('center_axis',(0.,0.,1.));
#16919=DIRECTION('ref_axis',(1.,0.,0.));
#16920=DIRECTION('',(0.,0.,-1.));
#16921=DIRECTION('center_axis',(0.,0.,1.));
#16922=DIRECTION('ref_axis',(1.,0.,0.));
#16923=DIRECTION('',(0.,0.,1.));
#16924=DIRECTION('center_axis',(0.,0.,1.));
#16925=DIRECTION('ref_axis',(1.,0.,0.));
#16926=DIRECTION('center_axis',(0.,0.,1.));
#16927=DIRECTION('ref_axis',(1.,0.,0.));
#16928=DIRECTION('center_axis',(0.,0.,1.));
#16929=DIRECTION('ref_axis',(1.,0.,0.));
#16930=DIRECTION('center_axis',(0.,0.,1.));
#16931=DIRECTION('ref_axis',(-0.707106781186548,-0.707106781186547,0.));
#16932=DIRECTION('',(0.,0.,-1.));
#16933=DIRECTION('center_axis',(0.,0.,1.));
#16934=DIRECTION('ref_axis',(1.,0.,0.));
#16935=DIRECTION('',(0.,0.,1.));
#16936=DIRECTION('center_axis',(0.,0.,1.));
#16937=DIRECTION('ref_axis',(1.,0.,0.));
#16938=DIRECTION('center_axis',(0.,0.,1.));
#16939=DIRECTION('ref_axis',(1.,0.,0.));
#16940=DIRECTION('center_axis',(0.,0.,1.));
#16941=DIRECTION('ref_axis',(1.,0.,0.));
#16942=DIRECTION('center_axis',(0.,0.,1.));
#16943=DIRECTION('ref_axis',(-0.707106781186547,0.707106781186548,0.));
#16944=DIRECTION('',(0.,0.,-1.));
#16945=DIRECTION('center_axis',(0.,0.,1.));
#16946=DIRECTION('ref_axis',(1.,0.,0.));
#16947=DIRECTION('',(0.,0.,1.));
#16948=DIRECTION('center_axis',(0.,0.,1.));
#16949=DIRECTION('ref_axis',(1.,0.,0.));
#16950=DIRECTION('center_axis',(0.,0.,1.));
#16951=DIRECTION('ref_axis',(1.,0.,0.));
#16952=DIRECTION('center_axis',(0.,0.,1.));
#16953=DIRECTION('ref_axis',(1.,0.,0.));
#16954=DIRECTION('center_axis',(0.,0.,1.));
#16955=DIRECTION('ref_axis',(1.,0.,0.));
#16956=DIRECTION('center_axis',(0.,0.,1.));
#16957=DIRECTION('ref_axis',(1.,0.,0.));
#16958=DIRECTION('',(0.,0.,1.));
#16959=DIRECTION('center_axis',(0.,0.,-1.));
#16960=DIRECTION('ref_axis',(1.,0.,0.));
#16961=DIRECTION('center_axis',(0.,0.,1.));
#16962=DIRECTION('ref_axis',(1.,0.,0.));
#16963=DIRECTION('center_axis',(0.,0.,1.));
#16964=DIRECTION('ref_axis',(1.,0.,0.));
#16965=DIRECTION('center_axis',(0.,0.,1.));
#16966=DIRECTION('ref_axis',(1.,0.,0.));
#16967=DIRECTION('center_axis',(0.,0.,1.));
#16968=DIRECTION('ref_axis',(1.,0.,0.));
#16969=DIRECTION('center_axis',(0.,0.,1.));
#16970=DIRECTION('ref_axis',(1.,0.,0.));
#16971=DIRECTION('center_axis',(0.,0.,1.));
#16972=DIRECTION('ref_axis',(1.,0.,0.));
#16973=DIRECTION('center_axis',(0.,0.,1.));
#16974=DIRECTION('ref_axis',(1.,0.,0.));
#16975=DIRECTION('center_axis',(0.,0.,-1.));
#16976=DIRECTION('ref_axis',(1.,0.,0.));
#16977=DIRECTION('center_axis',(0.,0.,-1.));
#16978=DIRECTION('ref_axis',(1.,0.,0.));
#16979=DIRECTION('center_axis',(0.,0.,-1.));
#16980=DIRECTION('ref_axis',(1.,0.,0.));
#16981=DIRECTION('center_axis',(0.,0.,1.));
#16982=DIRECTION('ref_axis',(1.,0.,0.));
#16983=DIRECTION('center_axis',(0.,0.,1.));
#16984=DIRECTION('ref_axis',(1.,0.,0.));
#16985=DIRECTION('',(0.,0.,1.));
#16986=DIRECTION('center_axis',(0.,0.,1.));
#16987=DIRECTION('ref_axis',(1.,0.,0.));
#16988=DIRECTION('center_axis',(0.,0.,1.));
#16989=DIRECTION('ref_axis',(1.,0.,0.));
#16990=DIRECTION('',(0.,0.,1.));
#16991=DIRECTION('center_axis',(0.,0.,1.));
#16992=DIRECTION('ref_axis',(1.,0.,0.));
#16993=DIRECTION('center_axis',(0.,0.,1.));
#16994=DIRECTION('ref_axis',(1.,0.,0.));
#16995=DIRECTION('',(0.,0.,1.));
#16996=DIRECTION('center_axis',(0.,0.,1.));
#16997=DIRECTION('ref_axis',(1.,0.,0.));
#16998=DIRECTION('center_axis',(0.,0.,1.));
#16999=DIRECTION('ref_axis',(1.,0.,0.));
#17000=DIRECTION('',(0.,0.,-1.));
#17001=DIRECTION('center_axis',(0.,0.,1.));
#17002=DIRECTION('ref_axis',(1.,0.,0.));
#17003=DIRECTION('center_axis',(0.,0.,1.));
#17004=DIRECTION('ref_axis',(1.,0.,0.));
#17005=DIRECTION('',(0.,0.,1.));
#17006=DIRECTION('center_axis',(0.,0.,-1.));
#17007=DIRECTION('ref_axis',(1.,0.,0.));
#17008=DIRECTION('center_axis',(0.,0.,1.));
#17009=DIRECTION('ref_axis',(1.,0.,0.));
#17010=DIRECTION('center_axis',(0.,0.,1.));
#17011=DIRECTION('ref_axis',(1.,0.,0.));
#17012=DIRECTION('center_axis',(0.,0.,1.));
#17013=DIRECTION('ref_axis',(1.,0.,0.));
#17014=DIRECTION('',(0.,0.,-1.));
#17015=DIRECTION('center_axis',(0.,0.,1.));
#17016=DIRECTION('ref_axis',(1.,0.,0.));
#17017=DIRECTION('center_axis',(0.,0.,1.));
#17018=DIRECTION('ref_axis',(1.,0.,0.));
#17019=DIRECTION('',(0.,0.,-1.));
#17020=DIRECTION('center_axis',(0.,0.,-1.));
#17021=DIRECTION('ref_axis',(1.,0.,0.));
#17022=DIRECTION('center_axis',(0.,0.,1.));
#17023=DIRECTION('ref_axis',(1.,0.,0.));
#17024=DIRECTION('center_axis',(0.,0.,1.));
#17025=DIRECTION('ref_axis',(1.,0.,0.));
#20782=CARTESIAN_POINT('',(0.,0.,0.));
#20783=CARTESIAN_POINT('Origin',(7.4,0.,5.4));
#20784=CARTESIAN_POINT('',(7.58034806292791,0.25,5.4));
#20785=CARTESIAN_POINT('',(7.6,2.03914977042615E-18,5.65));
#20786=CARTESIAN_POINT('Ctrl Pts',(7.58034806292791,0.25,5.4));
#20787=CARTESIAN_POINT('Ctrl Pts',(7.58034806292791,0.25,5.43144629923968));
#20788=CARTESIAN_POINT('Ctrl Pts',(7.58138367708303,0.243704881963377,5.46495278889766));
#20789=CARTESIAN_POINT('Ctrl Pts',(7.58510750685637,0.218175602614713,5.52653198325384));
#20790=CARTESIAN_POINT('Ctrl Pts',(7.58774011537305,0.198944206314965,5.55460918427831));
#20791=CARTESIAN_POINT('Ctrl Pts',(7.59266861270428,0.154609640177667,5.59894375041561));
#20792=CARTESIAN_POINT('Ctrl Pts',(7.59528712723235,0.126532242805987,5.61817550434358));
#20793=CARTESIAN_POINT('Ctrl Pts',(7.59897861635347,0.0649523762998013,
5.64370504368363));
#20794=CARTESIAN_POINT('Ctrl Pts',(7.6,0.0314456525117888,5.65));
#20795=CARTESIAN_POINT('Ctrl Pts',(7.6,2.77555756156289E-17,5.65));
#20796=CARTESIAN_POINT('Ctrl Pts',(7.6,3.46944695195361E-17,5.65));
#20797=CARTESIAN_POINT('Ctrl Pts',(7.6,-0.0314456525117888,5.65));
#20798=CARTESIAN_POINT('Ctrl Pts',(7.59897861635347,-0.0649523762997998,
5.64370504368363));
#20799=CARTESIAN_POINT('Ctrl Pts',(7.59528712723235,-0.126532242805986,
5.61817550434358));
#20800=CARTESIAN_POINT('Ctrl Pts',(7.59266861270428,-0.154609640177666,
5.59894375041561));
#20801=CARTESIAN_POINT('Ctrl Pts',(7.58774011537305,-0.198944206314964,
5.55460918427831));
#20802=CARTESIAN_POINT('Ctrl Pts',(7.58510750685637,-0.218175602614713,
5.52653198325384));
#20803=CARTESIAN_POINT('Ctrl Pts',(7.58138367708303,-0.243704881963377,
5.46495278889766));
#20804=CARTESIAN_POINT('Ctrl Pts',(7.58034806292791,-0.25,5.43144629923968));
#20805=CARTESIAN_POINT('Ctrl Pts',(7.58034806292791,-0.25,5.36855370076032));
#20806=CARTESIAN_POINT('Ctrl Pts',(7.58138367708303,-0.243704881963377,
5.33504721110235));
#20807=CARTESIAN_POINT('Ctrl Pts',(7.58510750685637,-0.218175602614713,
5.27346801674616));
#20808=CARTESIAN_POINT('Ctrl Pts',(7.58774011537305,-0.198944206314965,
5.24539081572169));
#20809=CARTESIAN_POINT('Ctrl Pts',(7.59266861270428,-0.154609640177667,
5.20105624958439));
#20810=CARTESIAN_POINT('Ctrl Pts',(7.59528712723235,-0.126532242805987,
5.18182449565642));
#20811=CARTESIAN_POINT('Ctrl Pts',(7.59897861635347,-0.0649523762998006,
5.15629495631637));
#20812=CARTESIAN_POINT('Ctrl Pts',(7.6,-0.0314456525117888,5.15));
#20813=CARTESIAN_POINT('Ctrl Pts',(7.6,0.0314456525117887,5.15));
#20814=CARTESIAN_POINT('Ctrl Pts',(7.59897861635347,0.0649523762998006,
5.15629495631637));
#20815=CARTESIAN_POINT('Ctrl Pts',(7.59528712723235,0.126532242805986,5.18182449565642));
#20816=CARTESIAN_POINT('Ctrl Pts',(7.59266861270428,0.154609640177666,5.20105624958439));
#20817=CARTESIAN_POINT('Ctrl Pts',(7.58774011537305,0.198944206314964,5.24539081572169));
#20818=CARTESIAN_POINT('Ctrl Pts',(7.58510750685637,0.218175602614713,5.27346801674616));
#20819=CARTESIAN_POINT('Ctrl Pts',(7.58138367708303,0.243704881963377,5.33504721110235));
#20820=CARTESIAN_POINT('Ctrl Pts',(7.58034806292791,0.25,5.36855370076032));
#20821=CARTESIAN_POINT('Ctrl Pts',(7.58034806292791,0.25,5.4));
#20822=CARTESIAN_POINT('',(9.,-3.06161699786838E-17,5.65));
#20823=CARTESIAN_POINT('',(7.4,-3.06161699786838E-17,5.65));
#20824=CARTESIAN_POINT('',(8.98956518577535,0.25,5.4));
#20825=CARTESIAN_POINT('Ctrl Pts',(8.98956518577535,0.25,5.4));
#20826=CARTESIAN_POINT('Ctrl Pts',(8.98956518577535,0.25,5.36859378633187));
#20827=CARTESIAN_POINT('Ctrl Pts',(8.99011104995181,0.24372047740942,5.33510417960069));
#20828=CARTESIAN_POINT('Ctrl Pts',(8.99208145165098,0.218202539734559,5.27351367328886));
#20829=CARTESIAN_POINT('Ctrl Pts',(8.99347740802958,0.198964922639276,5.245411532046));
#20830=CARTESIAN_POINT('Ctrl Pts',(8.99609686518216,0.154588504271054,5.20103511367778));
#20831=CARTESIAN_POINT('Ctrl Pts',(8.99749070376198,0.126486346986081,5.18179746841036));
#20832=CARTESIAN_POINT('Ctrl Pts',(8.99945625936844,0.0648957875009215,
5.15627950921557));
#20833=CARTESIAN_POINT('Ctrl Pts',(9.,0.0314061622633416,5.15));
#20834=CARTESIAN_POINT('Ctrl Pts',(9.,-0.0314061622633416,5.15));
#20835=CARTESIAN_POINT('Ctrl Pts',(8.99945625936844,-0.064895787500922,
5.15627950921557));
#20836=CARTESIAN_POINT('Ctrl Pts',(8.99749070376198,-0.126486346986081,
5.18179746841036));
#20837=CARTESIAN_POINT('Ctrl Pts',(8.99609686518216,-0.154588504271054,
5.20103511367778));
#20838=CARTESIAN_POINT('Ctrl Pts',(8.99347740802958,-0.198964922639276,
5.245411532046));
#20839=CARTESIAN_POINT('Ctrl Pts',(8.99208145165098,-0.218202539734559,
5.27351367328886));
#20840=CARTESIAN_POINT('Ctrl Pts',(8.99011104995181,-0.24372047740942,5.33510417960069));
#20841=CARTESIAN_POINT('Ctrl Pts',(8.98956518577535,-0.25,5.36859378633187));
#20842=CARTESIAN_POINT('Ctrl Pts',(8.98956518577535,-0.25,5.43140621366814));
#20843=CARTESIAN_POINT('Ctrl Pts',(8.99011104995181,-0.24372047740942,5.46489582039931));
#20844=CARTESIAN_POINT('Ctrl Pts',(8.99208145165098,-0.218202539734559,
5.52648632671114));
#20845=CARTESIAN_POINT('Ctrl Pts',(8.99347740802958,-0.198964922639276,
5.554588467954));
#20846=CARTESIAN_POINT('Ctrl Pts',(8.99609686518216,-0.154588504271054,
5.59896488632222));
#20847=CARTESIAN_POINT('Ctrl Pts',(8.99749070376198,-0.126486346986082,
5.61820253158964));
#20848=CARTESIAN_POINT('Ctrl Pts',(8.99945625936844,-0.0648957875009222,
5.64372049078443));
#20849=CARTESIAN_POINT('Ctrl Pts',(9.,-0.0314061622633417,5.65));
#20850=CARTESIAN_POINT('Ctrl Pts',(9.,-4.16333634234434E-17,5.65));
#20851=CARTESIAN_POINT('Ctrl Pts',(9.,-1.38777878078145E-17,5.65));
#20852=CARTESIAN_POINT('Ctrl Pts',(9.,0.0314061622633417,5.65));
#20853=CARTESIAN_POINT('Ctrl Pts',(8.99945625936844,0.0648957875009221,
5.64372049078443));
#20854=CARTESIAN_POINT('Ctrl Pts',(8.99749070376198,0.126486346986081,5.61820253158964));
#20855=CARTESIAN_POINT('Ctrl Pts',(8.99609686518216,0.154588504271054,5.59896488632222));
#20856=CARTESIAN_POINT('Ctrl Pts',(8.99347740802958,0.198964922639276,5.554588467954));
#20857=CARTESIAN_POINT('Ctrl Pts',(8.99208145165098,0.218202539734559,5.52648632671114));
#20858=CARTESIAN_POINT('Ctrl Pts',(8.99011104995181,0.24372047740942,5.46489582039931));
#20859=CARTESIAN_POINT('Ctrl Pts',(8.98956518577535,0.25,5.43140621366814));
#20860=CARTESIAN_POINT('Ctrl Pts',(8.98956518577535,0.25,5.4));
#20861=CARTESIAN_POINT('Origin',(4.05545635173699,-1.94454364826301,8.5));
#20862=CARTESIAN_POINT('',(3.89045635173699,-1.94454364826301,8.5));
#20863=CARTESIAN_POINT('Origin',(4.05545635173699,-1.94454364826301,8.5));
#20864=CARTESIAN_POINT('',(3.89045635173699,-1.94454364826301,9.2));
#20865=CARTESIAN_POINT('',(3.89045635173699,-1.94454364826301,8.5));
#20866=CARTESIAN_POINT('Origin',(4.05545635173699,-1.94454364826301,9.2));
#20867=CARTESIAN_POINT('Origin',(4.05545635173699,-1.94454364826301,8.5));
#20868=CARTESIAN_POINT('Origin',(4.05545635173699,1.94454364826301,8.5));
#20869=CARTESIAN_POINT('',(3.89045635173699,1.94454364826301,8.5));
#20870=CARTESIAN_POINT('Origin',(4.05545635173699,1.94454364826301,8.5));
#20871=CARTESIAN_POINT('',(3.89045635173699,1.94454364826301,9.2));
#20872=CARTESIAN_POINT('',(3.89045635173699,1.94454364826301,8.5));
#20873=CARTESIAN_POINT('Origin',(4.05545635173699,1.94454364826301,9.2));
#20874=CARTESIAN_POINT('Origin',(4.05545635173699,1.94454364826301,8.5));
#20875=CARTESIAN_POINT('Origin',(7.94454364826301,1.94454364826301,8.5));
#20876=CARTESIAN_POINT('',(7.77954364826301,1.94454364826301,8.5));
#20877=CARTESIAN_POINT('Origin',(7.94454364826301,1.94454364826301,8.5));
#20878=CARTESIAN_POINT('',(7.77954364826301,1.94454364826301,9.2));
#20879=CARTESIAN_POINT('',(7.77954364826301,1.94454364826301,8.5));
#20880=CARTESIAN_POINT('Origin',(7.94454364826301,1.94454364826301,9.2));
#20881=CARTESIAN_POINT('Origin',(7.94454364826301,1.94454364826301,8.5));
#20882=CARTESIAN_POINT('Origin',(7.944543648263,-1.94454364826301,8.5));
#20883=CARTESIAN_POINT('',(7.779543648263,-1.94454364826301,8.5));
#20884=CARTESIAN_POINT('Origin',(7.944543648263,-1.94454364826301,8.5));
#20885=CARTESIAN_POINT('',(7.779543648263,-1.94454364826301,9.2));
#20886=CARTESIAN_POINT('',(7.779543648263,-1.94454364826301,8.5));
#20887=CARTESIAN_POINT('Origin',(7.944543648263,-1.94454364826301,9.2));
#20888=CARTESIAN_POINT('Origin',(7.944543648263,-1.94454364826301,8.5));
#20889=CARTESIAN_POINT('Origin',(3.8079689783217,-2.1920310216783,4.));
#20890=CARTESIAN_POINT('',(4.2662001344149,-2.44825203483977,4.6));
#20891=CARTESIAN_POINT('',(4.2662001344149,-2.44825203483977,4.));
#20892=CARTESIAN_POINT('',(4.2662001344149,-2.44825203483977,4.));
#20893=CARTESIAN_POINT('',(3.55174796516023,-1.7337998655851,4.6));
#20894=CARTESIAN_POINT('Origin',(3.8079689783217,-2.1920310216783,4.6));
#20895=CARTESIAN_POINT('',(3.55174796516023,-1.7337998655851,4.));
#20896=CARTESIAN_POINT('',(3.55174796516023,-1.7337998655851,4.));
#20897=CARTESIAN_POINT('Origin',(3.8079689783217,-2.1920310216783,4.));
#20898=CARTESIAN_POINT('Origin',(3.8079689783217,-2.1920310216783,4.6));
#20899=CARTESIAN_POINT('Origin',(6.,0.,4.6));
#20900=CARTESIAN_POINT('Origin',(3.8079689783217,2.1920310216783,4.));
#20901=CARTESIAN_POINT('',(3.55174796516023,1.7337998655851,4.6));
#20902=CARTESIAN_POINT('',(3.55174796516023,1.7337998655851,4.));
#20903=CARTESIAN_POINT('',(3.55174796516023,1.7337998655851,4.));
#20904=CARTESIAN_POINT('',(4.2662001344149,2.44825203483977,4.6));
#20905=CARTESIAN_POINT('Origin',(3.8079689783217,2.1920310216783,4.6));
#20906=CARTESIAN_POINT('',(4.2662001344149,2.44825203483977,4.));
#20907=CARTESIAN_POINT('',(4.2662001344149,2.44825203483977,4.));
#20908=CARTESIAN_POINT('Origin',(3.8079689783217,2.1920310216783,4.));
#20909=CARTESIAN_POINT('Origin',(3.8079689783217,2.1920310216783,4.6));
#20910=CARTESIAN_POINT('Origin',(6.,0.,4.6));
#20911=CARTESIAN_POINT('Origin',(8.1920310216783,2.1920310216783,4.));
#20912=CARTESIAN_POINT('',(7.7337998655851,2.44825203483977,4.6));
#20913=CARTESIAN_POINT('',(7.7337998655851,2.44825203483977,4.));
#20914=CARTESIAN_POINT('',(7.7337998655851,2.44825203483977,4.));
#20915=CARTESIAN_POINT('',(8.44825203483977,1.7337998655851,4.6));
#20916=CARTESIAN_POINT('Origin',(8.1920310216783,2.1920310216783,4.6));
#20917=CARTESIAN_POINT('',(8.44825203483977,1.7337998655851,4.));
#20918=CARTESIAN_POINT('',(8.44825203483977,1.7337998655851,4.));
#20919=CARTESIAN_POINT('Origin',(8.1920310216783,2.1920310216783,4.));
#20920=CARTESIAN_POINT('Origin',(8.1920310216783,2.1920310216783,4.6));
#20921=CARTESIAN_POINT('Origin',(6.,0.,4.6));
#20922=CARTESIAN_POINT('Origin',(8.1920310216783,-2.1920310216783,4.));
#20923=CARTESIAN_POINT('',(8.44825203483977,-1.7337998655851,4.6));
#20924=CARTESIAN_POINT('',(8.44825203483977,-1.7337998655851,4.));
#20925=CARTESIAN_POINT('',(8.44825203483977,-1.7337998655851,4.));
#20926=CARTESIAN_POINT('',(7.7337998655851,-2.44825203483977,4.6));
#20927=CARTESIAN_POINT('Origin',(8.1920310216783,-2.1920310216783,4.6));
#20928=CARTESIAN_POINT('',(7.7337998655851,-2.44825203483977,4.));
#20929=CARTESIAN_POINT('',(7.7337998655851,-2.44825203483977,4.));
#20930=CARTESIAN_POINT('Origin',(8.1920310216783,-2.1920310216783,4.));
#20931=CARTESIAN_POINT('Origin',(8.1920310216783,-2.1920310216783,4.6));
#20932=CARTESIAN_POINT('Origin',(6.,0.,4.6));
#20933=CARTESIAN_POINT('Origin',(8.1920310216783,2.1920310216783,3.1));
#20934=CARTESIAN_POINT('',(7.9170310216783,2.1920310216783,3.2));
#20935=CARTESIAN_POINT('Origin',(8.1920310216783,2.1920310216783,3.2));
#20936=CARTESIAN_POINT('',(7.9170310216783,2.1920310216783,4.));
#20937=CARTESIAN_POINT('',(7.9170310216783,2.1920310216783,3.1));
#20938=CARTESIAN_POINT('Origin',(8.1920310216783,2.1920310216783,4.));
#20939=CARTESIAN_POINT('Origin',(6.,0.,4.));
#20940=CARTESIAN_POINT('',(2.5,-4.28626379701574E-16,4.));
#20941=CARTESIAN_POINT('Origin',(6.,0.,4.));
#20942=CARTESIAN_POINT('',(3.,-3.67394039744206E-16,4.));
#20943=CARTESIAN_POINT('Origin',(6.,0.,4.));
#20944=CARTESIAN_POINT('Origin',(6.,0.,4.));
#20945=CARTESIAN_POINT('Origin',(6.,0.,4.));
#20946=CARTESIAN_POINT('Origin',(6.,0.,4.));
#20947=CARTESIAN_POINT('Origin',(6.,0.,4.));
#20948=CARTESIAN_POINT('',(3.5329689783217,-2.1920310216783,4.));
#20949=CARTESIAN_POINT('Origin',(3.8079689783217,-2.1920310216783,4.));
#20950=CARTESIAN_POINT('',(7.9170310216783,-2.1920310216783,4.));
#20951=CARTESIAN_POINT('Origin',(8.1920310216783,-2.1920310216783,4.));
#20952=CARTESIAN_POINT('',(3.5329689783217,2.1920310216783,4.));
#20953=CARTESIAN_POINT('Origin',(3.8079689783217,2.1920310216783,4.));
#20954=CARTESIAN_POINT('Origin',(8.1920310216783,-2.1920310216783,3.1));
#20955=CARTESIAN_POINT('',(7.9170310216783,-2.1920310216783,3.2));
#20956=CARTESIAN_POINT('Origin',(8.1920310216783,-2.1920310216783,3.2));
#20957=CARTESIAN_POINT('',(7.9170310216783,-2.1920310216783,3.1));
#20958=CARTESIAN_POINT('Origin',(3.8079689783217,-2.1920310216783,3.1));
#20959=CARTESIAN_POINT('',(3.5329689783217,-2.1920310216783,3.2));
#20960=CARTESIAN_POINT('Origin',(3.8079689783217,-2.1920310216783,3.2));
#20961=CARTESIAN_POINT('',(3.5329689783217,-2.1920310216783,3.1));
#20962=CARTESIAN_POINT('Origin',(3.8079689783217,2.1920310216783,3.1));
#20963=CARTESIAN_POINT('',(3.5329689783217,2.1920310216783,3.2));
#20964=CARTESIAN_POINT('Origin',(3.8079689783217,2.1920310216783,3.2));
#20965=CARTESIAN_POINT('',(3.5329689783217,2.1920310216783,3.1));
#20966=CARTESIAN_POINT('Origin',(6.,0.,3.2));
#20967=CARTESIAN_POINT('',(3.,-3.67394039744206E-16,9.2));
#20968=CARTESIAN_POINT('Origin',(6.,0.,9.2));
#20969=CARTESIAN_POINT('',(3.,-3.67394039744206E-16,3.2));
#20970=CARTESIAN_POINT('Origin',(6.,0.,5.8));
#20971=CARTESIAN_POINT('',(3.65,-2.87791997799628E-16,5.8));
#20972=CARTESIAN_POINT('Origin',(6.,0.,5.8));
#20973=CARTESIAN_POINT('',(3.65,2.87791997799628E-16,9.2));
#20974=CARTESIAN_POINT('',(3.65,-2.87791997799628E-16,5.8));
#20975=CARTESIAN_POINT('Origin',(6.,0.,9.2));
#20976=CARTESIAN_POINT('Origin',(6.,0.,5.8));
#20977=CARTESIAN_POINT('',(4.4,-1.95943487863576E-16,5.8));
#20978=CARTESIAN_POINT('Origin',(6.,0.,5.8));
#20979=CARTESIAN_POINT('Origin',(6.,0.,3.2));
#20980=CARTESIAN_POINT('',(2.5,-4.28626379701574E-16,3.2));
#20981=CARTESIAN_POINT('',(2.5,-4.28626379701574E-16,3.2));
#20982=CARTESIAN_POINT('Origin',(6.,0.,3.2));
#20983=CARTESIAN_POINT('Origin',(6.,0.,3.2));
#20984=CARTESIAN_POINT('',(4.4,-1.95943487863576E-16,3.2));
#20985=CARTESIAN_POINT('',(4.4,-1.95943487863576E-16,3.2));
#20986=CARTESIAN_POINT('Origin',(6.,0.,3.2));
#20987=CARTESIAN_POINT('Origin',(6.,0.,9.2));
#20988=CARTESIAN_POINT('Origin',(6.,0.,3.2));
#57807=UNCERTAINTY_MEASURE_WITH_UNIT(LENGTH_MEASURE(0.001),#57901,
'DISTANCE_ACCURACY_VALUE',
'Maximum model space distance between geometric entities at asserted c
onnectivities');
#57841=UNCERTAINTY_MEASURE_WITH_UNIT(LENGTH_MEASURE(0.001),#57901,
'DISTANCE_ACCURACY_VALUE',
'Maximum model space distance between geometric entities at asserted c
onnectivities');
#57866=(
GEOMETRIC_REPRESENTATION_CONTEXT(3)
GLOBAL_UNCERTAINTY_ASSIGNED_CONTEXT((#57807))
GLOBAL_UNIT_ASSIGNED_CONTEXT((#57901,#57903,#57904))
REPRESENTATION_CONTEXT('','3D')
);
#57900=(
GEOMETRIC_REPRESENTATION_CONTEXT(3)
GLOBAL_UNCERTAINTY_ASSIGNED_CONTEXT((#57841))
GLOBAL_UNIT_ASSIGNED_CONTEXT((#57901,#57903,#57904))
REPRESENTATION_CONTEXT('','3D')
);
#57901=(
LENGTH_UNIT()
NAMED_UNIT(*)
SI_UNIT(.CENTI.,.METRE.)
);
#57903=(
NAMED_UNIT(*)
PLANE_ANGLE_UNIT()
SI_UNIT($,.RADIAN.)
);
#57904=(
NAMED_UNIT(*)
SI_UNIT($,.STERADIAN.)
SOLID_ANGLE_UNIT()
);
#57929=SHAPE_DEFINITION_REPRESENTATION(#57992,#58133);
#57992=PRODUCT_DEFINITION_SHAPE('',$,#58192);
#58133=SHAPE_REPRESENTATION('',(#14701),#57866);
#58167=PRODUCT_DEFINITION_CONTEXT('part definition',#58343,'design');
#58192=PRODUCT_DEFINITION('Output bearing post','Output bearing post',#58250,
#58167);
#58250=PRODUCT_DEFINITION_FORMATION('',$,#58369);
#58343=APPLICATION_CONTEXT(
'Core Data for Automotive Mechanical Design Process');
#58344=PRODUCT_CONTEXT('part definition',#58343,'mechanical');
#58369=PRODUCT('Output bearing post','Output bearing post',
'Output bearing post',(#58344));
#58459=COLOUR_RGB('Grey',0.48,0.52,0.57);
#58460=FILL_AREA_STYLE_COLOUR('',#58459);
#58461=FILL_AREA_STYLE('',(#58460));
#58462=SURFACE_STYLE_FILL_AREA(#58461);
#58463=SURFACE_SIDE_STYLE('',(#58462));
#58464=SURFACE_STYLE_USAGE(.BOTH.,#58463);
#58465=PRESENTATION_STYLE_ASSIGNMENT((#58464));
ENDSEC;
END-ISO-10303-21;
